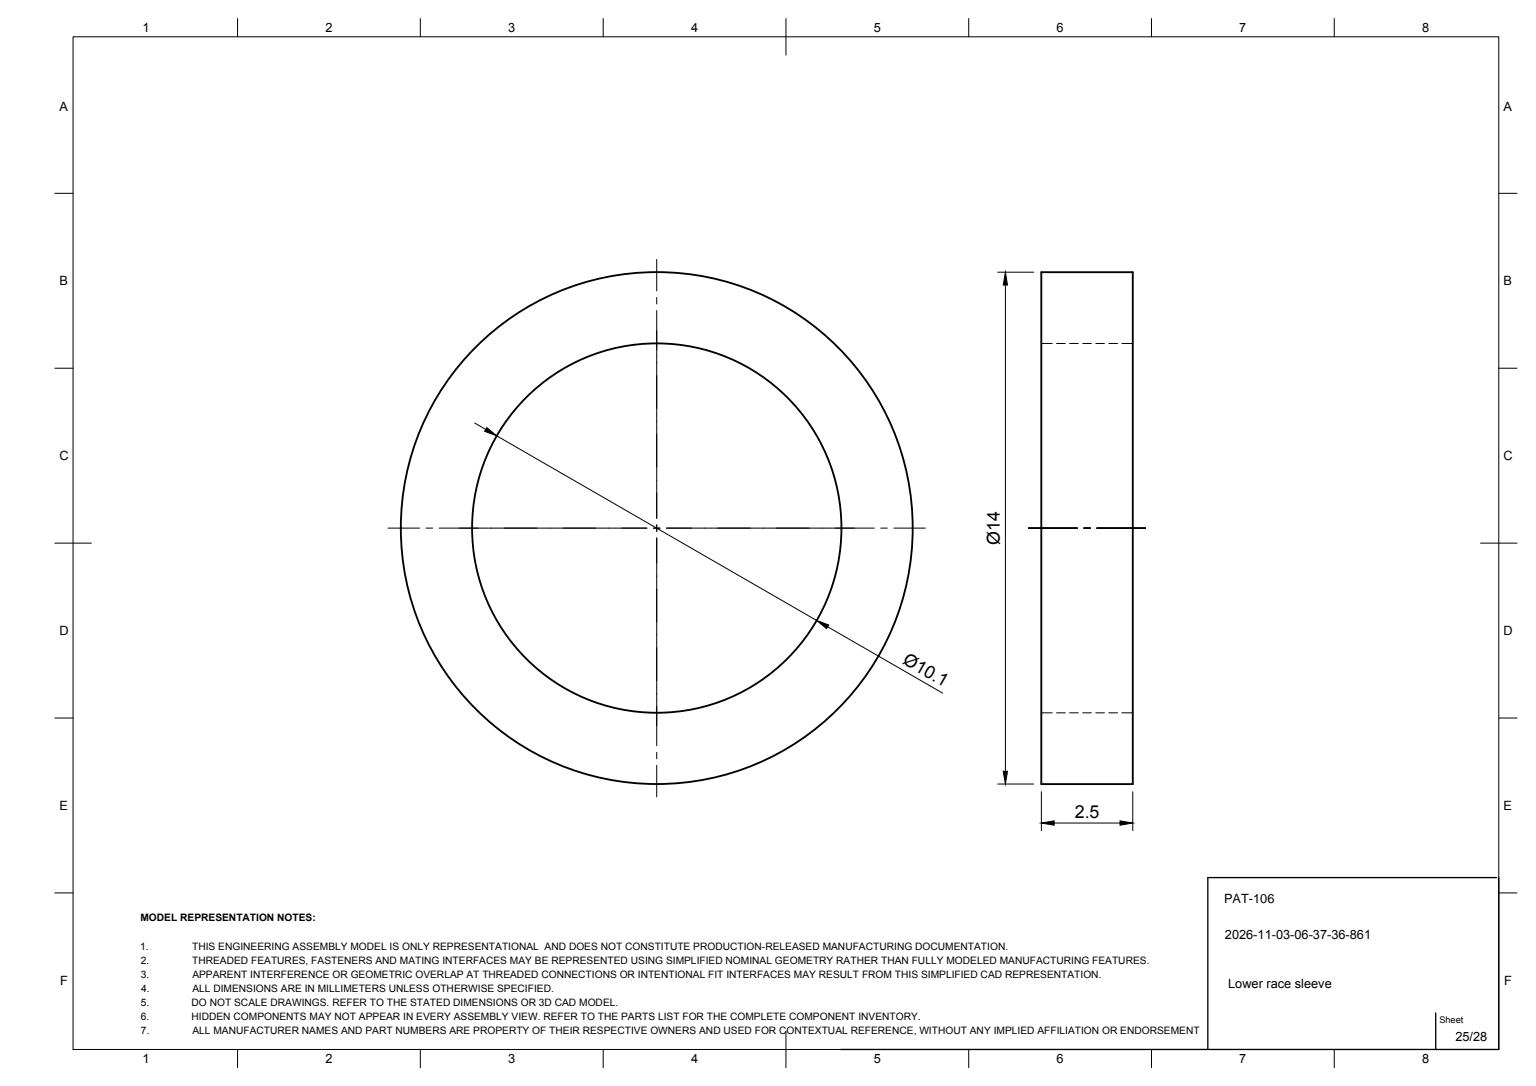
ISO-10303-21;
HEADER;
/* Generated by software containing ST-Developer
 * from STEP Tools, Inc. (www.steptools.com) 
 */

FILE_DESCRIPTION(
/* description */ ('Torsion-spring ratchet demonstrator'),
/* implementation_level */ '2;1');

FILE_NAME(
/* name */ 'Lower race sleeve.step',
/* time_stamp */ '2026-10-29T17:29:17-07:00',
/* author */ (''),
/* organization */ (''),
/* preprocessor_version */ 'ST-DEVELOPER v20.2',
/* originating_system */ 'Autodesk Translation Framework v15.17.0.0',
/* authorisation */ '');

FILE_SCHEMA (('AUTOMOTIVE_DESIGN { 1 0 10303 214 3 1 1 }'));
ENDSEC;

DATA;
#10=MECHANICAL_DESIGN_GEOMETRIC_PRESENTATION_REPRESENTATION('',(#309),#11258);
#253=SHAPE_REPRESENTATION_RELATIONSHIP('SRR','None',#11381,#277);
#277=ADVANCED_BREP_SHAPE_REPRESENTATION('',(#339),#11251);
#309=STYLED_ITEM('',(#11570),#339);
#339=MANIFOLD_SOLID_BREP('Body1',#5182);
#422=FACE_BOUND('',#1207,.T.);
#423=FACE_BOUND('',#1209,.T.);
#534=PLANE('',#5916);
#535=PLANE('',#5917);
#822=FACE_OUTER_BOUND('',#1204,.T.);
#823=FACE_OUTER_BOUND('',#1205,.T.);
#824=FACE_OUTER_BOUND('',#1206,.T.);
#825=FACE_OUTER_BOUND('',#1208,.T.);
#1204=EDGE_LOOP('',(#4230,#4231,#4232,#4233));
#1205=EDGE_LOOP('',(#4234,#4235,#4236,#4237));
#1206=EDGE_LOOP('',(#4238));
#1207=EDGE_LOOP('',(#4239));
#1208=EDGE_LOOP('',(#4240));
#1209=EDGE_LOOP('',(#4241));
#1484=LINE('',#10517,#1867);
#1485=LINE('',#10523,#1868);
#1867=VECTOR('',#7143,0.505);
#1868=VECTOR('',#7150,0.7);
#2301=CIRCLE('',#5911,0.505);
#2302=CIRCLE('',#5912,0.505);
#2303=CIRCLE('',#5914,0.7);
#2304=CIRCLE('',#5915,0.7);
#2605=VERTEX_POINT('',#10514);
#2606=VERTEX_POINT('',#10516);
#2607=VERTEX_POINT('',#10520);
#2608=VERTEX_POINT('',#10522);
#3175=EDGE_CURVE('',#2605,#2605,#2301,.T.);
#3176=EDGE_CURVE('',#2605,#2606,#1484,.T.);
#3177=EDGE_CURVE('',#2606,#2606,#2302,.T.);
#3178=EDGE_CURVE('',#2607,#2607,#2303,.T.);
#3179=EDGE_CURVE('',#2607,#2608,#1485,.T.);
#3180=EDGE_CURVE('',#2608,#2608,#2304,.T.);
#4230=ORIENTED_EDGE('',*,*,#3175,.F.);
#4231=ORIENTED_EDGE('',*,*,#3176,.T.);
#4232=ORIENTED_EDGE('',*,*,#3177,.T.);
#4233=ORIENTED_EDGE('',*,*,#3176,.F.);
#4234=ORIENTED_EDGE('',*,*,#3178,.F.);
#4235=ORIENTED_EDGE('',*,*,#3179,.T.);
#4236=ORIENTED_EDGE('',*,*,#3180,.T.);
#4237=ORIENTED_EDGE('',*,*,#3179,.F.);
#4238=ORIENTED_EDGE('',*,*,#3178,.T.);
#4239=ORIENTED_EDGE('',*,*,#3175,.T.);
#4240=ORIENTED_EDGE('',*,*,#3180,.F.);
#4241=ORIENTED_EDGE('',*,*,#3177,.F.);
#4835=CYLINDRICAL_SURFACE('',#5910,0.505);
#4836=CYLINDRICAL_SURFACE('',#5913,0.7);
#5048=ADVANCED_FACE('',(#822),#4835,.F.);
#5049=ADVANCED_FACE('',(#823),#4836,.T.);
#5050=ADVANCED_FACE('',(#824,#422),#534,.T.);
#5051=ADVANCED_FACE('',(#825,#423),#535,.F.);
#5182=CLOSED_SHELL('',(#5048,#5049,#5050,#5051));
#5909=AXIS2_PLACEMENT_3D('',#10512,#7137,#7138);
#5910=AXIS2_PLACEMENT_3D('',#10513,#7139,#7140);
#5911=AXIS2_PLACEMENT_3D('',#10515,#7141,#7142);
#5912=AXIS2_PLACEMENT_3D('',#10518,#7144,#7145);
#5913=AXIS2_PLACEMENT_3D('',#10519,#7146,#7147);
#5914=AXIS2_PLACEMENT_3D('',#10521,#7148,#7149);
#5915=AXIS2_PLACEMENT_3D('',#10524,#7151,#7152);
#5916=AXIS2_PLACEMENT_3D('',#10525,#7153,#7154);
#5917=AXIS2_PLACEMENT_3D('',#10526,#7155,#7156);
#7137=DIRECTION('axis',(0.,0.,1.));
#7138=DIRECTION('refdir',(1.,0.,0.));
#7139=DIRECTION('center_axis',(0.,0.,1.));
#7140=DIRECTION('ref_axis',(1.,0.,0.));
#7141=DIRECTION('center_axis',(0.,0.,-1.));
#7142=DIRECTION('ref_axis',(1.,0.,0.));
#7143=DIRECTION('',(0.,0.,-1.));
#7144=DIRECTION('center_axis',(0.,0.,-1.));
#7145=DIRECTION('ref_axis',(1.,0.,0.));
#7146=DIRECTION('center_axis',(0.,0.,1.));
#7147=DIRECTION('ref_axis',(1.,0.,0.));
#7148=DIRECTION('center_axis',(0.,0.,1.));
#7149=DIRECTION('ref_axis',(1.,0.,0.));
#7150=DIRECTION('',(0.,0.,-1.));
#7151=DIRECTION('center_axis',(0.,0.,1.));
#7152=DIRECTION('ref_axis',(1.,0.,0.));
#7153=DIRECTION('center_axis',(0.,0.,1.));
#7154=DIRECTION('ref_axis',(1.,0.,0.));
#7155=DIRECTION('center_axis',(0.,0.,1.));
#7156=DIRECTION('ref_axis',(1.,0.,0.));
#10512=CARTESIAN_POINT('',(0.,0.,0.));
#10513=CARTESIAN_POINT('Origin',(0.,0.,1.8));
#10514=CARTESIAN_POINT('',(-0.505,-6.18446633569413E-17,2.05));
#10515=CARTESIAN_POINT('Origin',(0.,0.,2.05));
#10516=CARTESIAN_POINT('',(-0.505,-6.18446633569413E-17,1.8));
#10517=CARTESIAN_POINT('',(-0.505,-6.18446633569413E-17,1.8));
#10518=CARTESIAN_POINT('Origin',(0.,0.,1.8));
#10519=CARTESIAN_POINT('Origin',(0.,0.,1.8));
#10520=CARTESIAN_POINT('',(-0.7,-8.57252759403147E-17,2.05));
#10521=CARTESIAN_POINT('Origin',(0.,0.,2.05));
#10522=CARTESIAN_POINT('',(-0.7,-8.57252759403147E-17,1.8));
#10523=CARTESIAN_POINT('',(-0.7,-8.57252759403147E-17,1.8));
#10524=CARTESIAN_POINT('Origin',(0.,0.,1.8));
#10525=CARTESIAN_POINT('Origin',(0.,0.,2.05));
#10526=CARTESIAN_POINT('Origin',(0.,0.,1.8));
#11221=UNCERTAINTY_MEASURE_WITH_UNIT(LENGTH_MEASURE(0.001),#11259,
'DISTANCE_ACCURACY_VALUE',
'Maximum model space distance between geometric entities at asserted c
onnectivities');
#11228=UNCERTAINTY_MEASURE_WITH_UNIT(LENGTH_MEASURE(0.001),#11259,
'DISTANCE_ACCURACY_VALUE',
'Maximum model space distance between geometric entities at asserted c
onnectivities');
#11251=(
GEOMETRIC_REPRESENTATION_CONTEXT(3)
GLOBAL_UNCERTAINTY_ASSIGNED_CONTEXT((#11221))
GLOBAL_UNIT_ASSIGNED_CONTEXT((#11259,#11261,#11262))
REPRESENTATION_CONTEXT('','3D')
);
#11258=(
GEOMETRIC_REPRESENTATION_CONTEXT(3)
GLOBAL_UNCERTAINTY_ASSIGNED_CONTEXT((#11228))
GLOBAL_UNIT_ASSIGNED_CONTEXT((#11259,#11261,#11262))
REPRESENTATION_CONTEXT('','3D')
);
#11259=(
LENGTH_UNIT()
NAMED_UNIT(*)
SI_UNIT(.CENTI.,.METRE.)
);
#11261=(
NAMED_UNIT(*)
PLANE_ANGLE_UNIT()
SI_UNIT($,.RADIAN.)
);
#11262=(
NAMED_UNIT(*)
SI_UNIT($,.STERADIAN.)
SOLID_ANGLE_UNIT()
);
#11285=SHAPE_DEFINITION_REPRESENTATION(#11342,#11381);
#11342=PRODUCT_DEFINITION_SHAPE('',$,#11411);
#11381=SHAPE_REPRESENTATION('',(#5909),#11251);
#11388=PRODUCT_DEFINITION_CONTEXT('part definition',#11477,'design');
#11411=PRODUCT_DEFINITION('Lower race sleeve','Lower race sleeve',#11440,
#11388);
#11440=PRODUCT_DEFINITION_FORMATION('',$,#11501);
#11477=APPLICATION_CONTEXT(
'Core Data for Automotive Mechanical Design Process');
#11478=PRODUCT_CONTEXT('part definition',#11477,'mechanical');
#11501=PRODUCT('Lower race sleeve','Lower race sleeve',
'Lower race sleeve',(#11478));
#11564=COLOUR_RGB('Light Blue',0.38,0.62,0.78);
#11565=FILL_AREA_STYLE_COLOUR('',#11564);
#11566=FILL_AREA_STYLE('',(#11565));
#11567=SURFACE_STYLE_FILL_AREA(#11566);
#11568=SURFACE_SIDE_STYLE('',(#11567));
#11569=SURFACE_STYLE_USAGE(.BOTH.,#11568);
#11570=PRESENTATION_STYLE_ASSIGNMENT((#11569));
ENDSEC;
END-ISO-10303-21;
